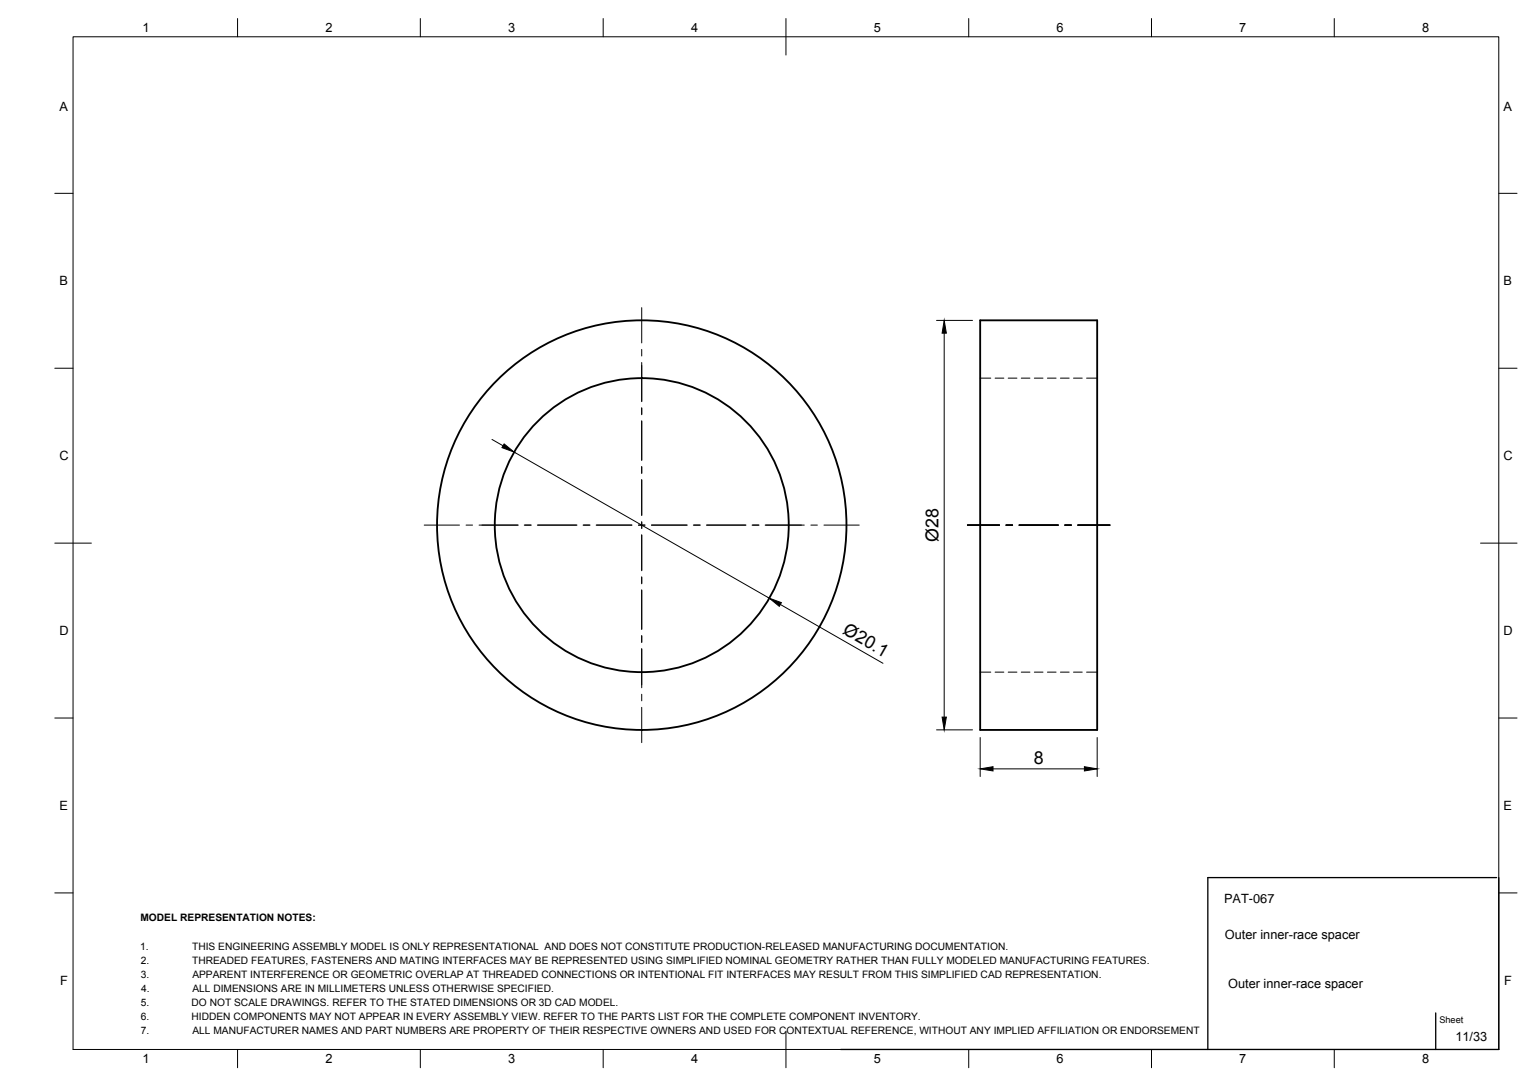
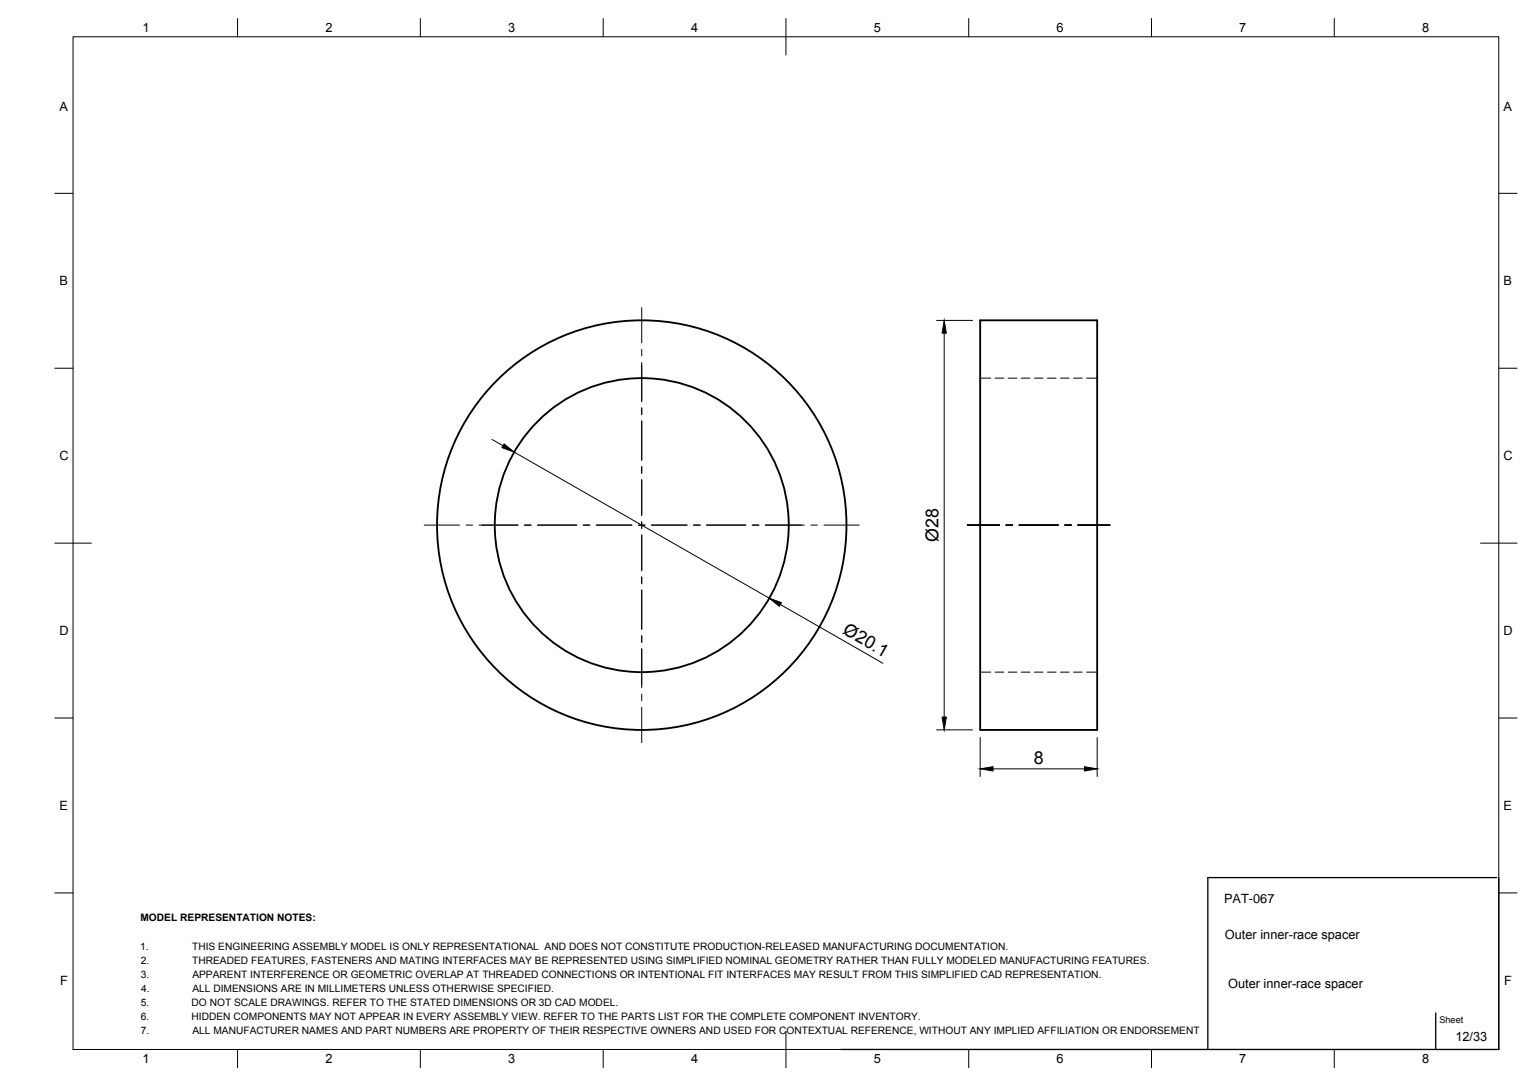
ISO-10303-21;
HEADER;
/* Generated by software containing ST-Developer
 * from STEP Tools, Inc. (www.steptools.com) 
 */

FILE_DESCRIPTION(
/* description */ ('Lifting hook block with sheave'),
/* implementation_level */ '2;1');

FILE_NAME(
/* name */ 'Outer inner-race spacer.step',
/* time_stamp */ '2026-10-28T03:23:54-07:00',
/* author */ (''),
/* organization */ (''),
/* preprocessor_version */ 'ST-DEVELOPER v20.2',
/* originating_system */ 'Autodesk Translation Framework v15.17.0.0',
/* authorisation */ '');

FILE_SCHEMA (('AUTOMOTIVE_DESIGN { 1 0 10303 214 3 1 1 }'));
ENDSEC;

DATA;
#10=MECHANICAL_DESIGN_GEOMETRIC_PRESENTATION_REPRESENTATION('',(#357),#9391);
#297=SHAPE_REPRESENTATION_RELATIONSHIP('SRR','None',#9528,#327);
#327=ADVANCED_BREP_SHAPE_REPRESENTATION('',(#395),#9363);
#357=STYLED_ITEM('',(#9745),#395);
#395=MANIFOLD_SOLID_BREP('Body1',#4893);
#528=LINE('',#7964,#816);
#529=LINE('',#7970,#817);
#816=VECTOR('',#6379,1.005);
#817=VECTOR('',#6386,1.4);
#1036=CYLINDRICAL_SURFACE('',#5430,1.005);
#1037=CYLINDRICAL_SURFACE('',#5433,1.4);
#1147=FACE_BOUND('',#1628,.T.);
#1148=FACE_BOUND('',#1630,.T.);
#1296=FACE_OUTER_BOUND('',#1625,.T.);
#1297=FACE_OUTER_BOUND('',#1626,.T.);
#1298=FACE_OUTER_BOUND('',#1627,.T.);
#1299=FACE_OUTER_BOUND('',#1629,.T.);
#1625=EDGE_LOOP('',(#3614,#3615,#3616,#3617));
#1626=EDGE_LOOP('',(#3618,#3619,#3620,#3621));
#1627=EDGE_LOOP('',(#3622));
#1628=EDGE_LOOP('',(#3623));
#1629=EDGE_LOOP('',(#3624));
#1630=EDGE_LOOP('',(#3625));
#2003=CIRCLE('',#5431,1.005);
#2004=CIRCLE('',#5432,1.005);
#2005=CIRCLE('',#5434,1.4);
#2006=CIRCLE('',#5435,1.4);
#2336=VERTEX_POINT('',#7961);
#2337=VERTEX_POINT('',#7963);
#2338=VERTEX_POINT('',#7967);
#2339=VERTEX_POINT('',#7969);
#2811=EDGE_CURVE('',#2336,#2336,#2003,.T.);
#2812=EDGE_CURVE('',#2336,#2337,#528,.T.);
#2813=EDGE_CURVE('',#2337,#2337,#2004,.T.);
#2814=EDGE_CURVE('',#2338,#2338,#2005,.T.);
#2815=EDGE_CURVE('',#2338,#2339,#529,.T.);
#2816=EDGE_CURVE('',#2339,#2339,#2006,.T.);
#3614=ORIENTED_EDGE('',*,*,#2811,.F.);
#3615=ORIENTED_EDGE('',*,*,#2812,.T.);
#3616=ORIENTED_EDGE('',*,*,#2813,.T.);
#3617=ORIENTED_EDGE('',*,*,#2812,.F.);
#3618=ORIENTED_EDGE('',*,*,#2814,.F.);
#3619=ORIENTED_EDGE('',*,*,#2815,.T.);
#3620=ORIENTED_EDGE('',*,*,#2816,.T.);
#3621=ORIENTED_EDGE('',*,*,#2815,.F.);
#3622=ORIENTED_EDGE('',*,*,#2814,.T.);
#3623=ORIENTED_EDGE('',*,*,#2811,.T.);
#3624=ORIENTED_EDGE('',*,*,#2816,.F.);
#3625=ORIENTED_EDGE('',*,*,#2813,.F.);
#4490=PLANE('',#5436);
#4491=PLANE('',#5437);
#4672=ADVANCED_FACE('',(#1296),#1036,.F.);
#4673=ADVANCED_FACE('',(#1297),#1037,.T.);
#4674=ADVANCED_FACE('',(#1298,#1147),#4490,.T.);
#4675=ADVANCED_FACE('',(#1299,#1148),#4491,.F.);
#4893=CLOSED_SHELL('',(#4672,#4673,#4674,#4675));
#5429=AXIS2_PLACEMENT_3D('',#7959,#6373,#6374);
#5430=AXIS2_PLACEMENT_3D('',#7960,#6375,#6376);
#5431=AXIS2_PLACEMENT_3D('',#7962,#6377,#6378);
#5432=AXIS2_PLACEMENT_3D('',#7965,#6380,#6381);
#5433=AXIS2_PLACEMENT_3D('',#7966,#6382,#6383);
#5434=AXIS2_PLACEMENT_3D('',#7968,#6384,#6385);
#5435=AXIS2_PLACEMENT_3D('',#7971,#6387,#6388);
#5436=AXIS2_PLACEMENT_3D('',#7972,#6389,#6390);
#5437=AXIS2_PLACEMENT_3D('',#7973,#6391,#6392);
#6373=DIRECTION('axis',(0.,0.,1.));
#6374=DIRECTION('refdir',(1.,0.,0.));
#6375=DIRECTION('center_axis',(0.,1.,0.));
#6376=DIRECTION('ref_axis',(1.,0.,0.));
#6377=DIRECTION('center_axis',(0.,-1.,0.));
#6378=DIRECTION('ref_axis',(1.,0.,0.));
#6379=DIRECTION('',(0.,-1.,0.));
#6380=DIRECTION('center_axis',(0.,-1.,0.));
#6381=DIRECTION('ref_axis',(1.,0.,0.));
#6382=DIRECTION('center_axis',(0.,1.,0.));
#6383=DIRECTION('ref_axis',(1.,0.,0.));
#6384=DIRECTION('center_axis',(0.,1.,0.));
#6385=DIRECTION('ref_axis',(1.,0.,0.));
#6386=DIRECTION('',(0.,-1.,0.));
#6387=DIRECTION('center_axis',(0.,1.,0.));
#6388=DIRECTION('ref_axis',(1.,0.,0.));
#6389=DIRECTION('center_axis',(0.,1.,0.));
#6390=DIRECTION('ref_axis',(1.,0.,0.));
#6391=DIRECTION('center_axis',(0.,1.,0.));
#6392=DIRECTION('ref_axis',(1.,0.,0.));
#7959=CARTESIAN_POINT('',(0.,0.,0.));
#7960=CARTESIAN_POINT('Origin',(0.,-2.5,12.));
#7961=CARTESIAN_POINT('',(-1.005,-1.7,12.));
#7962=CARTESIAN_POINT('Origin',(0.,-1.7,12.));
#7963=CARTESIAN_POINT('',(-1.005,-2.5,12.));
#7964=CARTESIAN_POINT('',(-1.005,-2.5,12.));
#7965=CARTESIAN_POINT('Origin',(0.,-2.5,12.));
#7966=CARTESIAN_POINT('Origin',(0.,-2.5,12.));
#7967=CARTESIAN_POINT('',(-1.4,-1.7,12.));
#7968=CARTESIAN_POINT('Origin',(0.,-1.7,12.));
#7969=CARTESIAN_POINT('',(-1.4,-2.5,12.));
#7970=CARTESIAN_POINT('',(-1.4,-2.5,12.));
#7971=CARTESIAN_POINT('Origin',(0.,-2.5,12.));
#7972=CARTESIAN_POINT('Origin',(0.,-1.7,12.));
#7973=CARTESIAN_POINT('Origin',(0.,-2.5,12.));
#9326=UNCERTAINTY_MEASURE_WITH_UNIT(LENGTH_MEASURE(0.001),#9392,
'DISTANCE_ACCURACY_VALUE',
'Maximum model space distance between geometric entities at asserted c
onnectivities');
#9354=UNCERTAINTY_MEASURE_WITH_UNIT(LENGTH_MEASURE(0.001),#9392,
'DISTANCE_ACCURACY_VALUE',
'Maximum model space distance between geometric entities at asserted c
onnectivities');
#9363=(
GEOMETRIC_REPRESENTATION_CONTEXT(3)
GLOBAL_UNCERTAINTY_ASSIGNED_CONTEXT((#9326))
GLOBAL_UNIT_ASSIGNED_CONTEXT((#9392,#9394,#9395))
REPRESENTATION_CONTEXT('','3D')
);
#9391=(
GEOMETRIC_REPRESENTATION_CONTEXT(3)
GLOBAL_UNCERTAINTY_ASSIGNED_CONTEXT((#9354))
GLOBAL_UNIT_ASSIGNED_CONTEXT((#9392,#9394,#9395))
REPRESENTATION_CONTEXT('','3D')
);
#9392=(
LENGTH_UNIT()
NAMED_UNIT(*)
SI_UNIT(.CENTI.,.METRE.)
);
#9394=(
NAMED_UNIT(*)
PLANE_ANGLE_UNIT()
SI_UNIT($,.RADIAN.)
);
#9395=(
NAMED_UNIT(*)
SI_UNIT($,.STERADIAN.)
SOLID_ANGLE_UNIT()
);
#9404=SHAPE_DEFINITION_REPRESENTATION(#9440,#9528);
#9440=PRODUCT_DEFINITION_SHAPE('',$,#9565);
#9528=SHAPE_REPRESENTATION('',(#5429),#9363);
#9556=PRODUCT_DEFINITION_CONTEXT('part definition',#9666,'design');
#9565=PRODUCT_DEFINITION('Outer inner-race spacer',
'Outer inner-race spacer',#9601,#9556);
#9601=PRODUCT_DEFINITION_FORMATION('',$,#9676);
#9666=APPLICATION_CONTEXT(
'Core Data for Automotive Mechanical Design Process');
#9667=PRODUCT_CONTEXT('part definition',#9666,'mechanical');
#9676=PRODUCT('Outer inner-race spacer','Outer inner-race spacer',
'Outer inner-race spacer',(#9667));
#9739=COLOUR_RGB('Light Blue',0.38,0.62,0.78);
#9740=FILL_AREA_STYLE_COLOUR('',#9739);
#9741=FILL_AREA_STYLE('',(#9740));
#9742=SURFACE_STYLE_FILL_AREA(#9741);
#9743=SURFACE_SIDE_STYLE('',(#9742));
#9744=SURFACE_STYLE_USAGE(.BOTH.,#9743);
#9745=PRESENTATION_STYLE_ASSIGNMENT((#9744));
ENDSEC;
END-ISO-10303-21;
